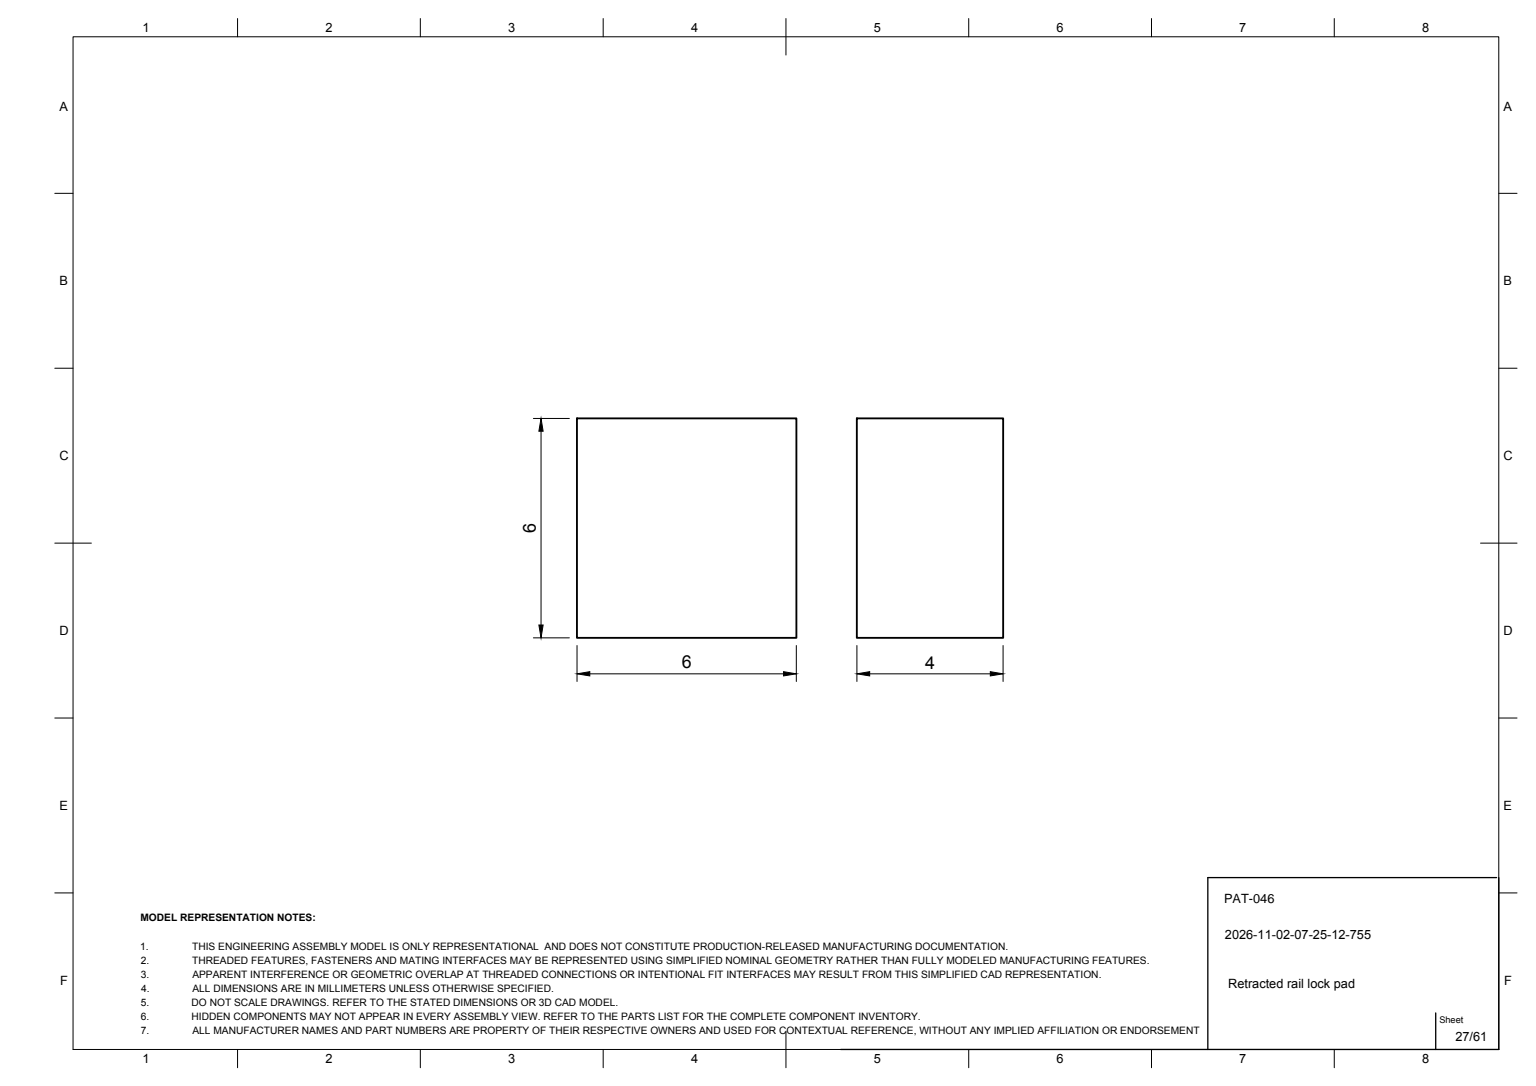
ISO-10303-21;
HEADER;
/* Generated by software containing ST-Developer
 * from STEP Tools, Inc. (www.steptools.com) 
 */

FILE_DESCRIPTION(
/* description */ ('Gear mesh backlash fixture'),
/* implementation_level */ '2;1');

FILE_NAME(
/* name */ 'Retracted rail lock pad.step',
/* time_stamp */ '2026-10-28T03:26:00-07:00',
/* author */ (''),
/* organization */ (''),
/* preprocessor_version */ 'ST-DEVELOPER v20.2',
/* originating_system */ 'Autodesk Translation Framework v15.17.0.0',
/* authorisation */ '');

FILE_SCHEMA (('AUTOMOTIVE_DESIGN { 1 0 10303 214 3 1 1 }'));
ENDSEC;

DATA;
#10=MECHANICAL_DESIGN_GEOMETRIC_PRESENTATION_REPRESENTATION('',(#1042),#57900);
#935=SHAPE_REPRESENTATION_RELATIONSHIP('SRR','None',#58132,#985);
#985=ADVANCED_BREP_SHAPE_REPRESENTATION('',(#1106),#57865);
#1042=STYLED_ITEM('',(#58479),#1106);
#1106=MANIFOLD_SOLID_BREP('Body1',#13603);
#1452=PLANE('',#14695);
#1453=PLANE('',#14696);
#1454=PLANE('',#14697);
#1455=PLANE('',#14698);
#1456=PLANE('',#14699);
#1457=PLANE('',#14700);
#1927=FACE_OUTER_BOUND('',#2795,.T.);
#1928=FACE_OUTER_BOUND('',#2796,.T.);
#1929=FACE_OUTER_BOUND('',#2797,.T.);
#1930=FACE_OUTER_BOUND('',#2798,.T.);
#1931=FACE_OUTER_BOUND('',#2799,.T.);
#1932=FACE_OUTER_BOUND('',#2800,.T.);
#2795=EDGE_LOOP('',(#9923,#9924,#9925,#9926));
#2796=EDGE_LOOP('',(#9927,#9928,#9929,#9930));
#2797=EDGE_LOOP('',(#9931,#9932,#9933,#9934));
#2798=EDGE_LOOP('',(#9935,#9936,#9937,#9938));
#2799=EDGE_LOOP('',(#9939,#9940,#9941,#9942));
#2800=EDGE_LOOP('',(#9943,#9944,#9945,#9946));
#3674=LINE('',#20759,#4563);
#3675=LINE('',#20761,#4564);
#3676=LINE('',#20763,#4565);
#3677=LINE('',#20764,#4566);
#3678=LINE('',#20767,#4567);
#3679=LINE('',#20769,#4568);
#3680=LINE('',#20770,#4569);
#3681=LINE('',#20773,#4570);
#3682=LINE('',#20775,#4571);
#3683=LINE('',#20776,#4572);
#3684=LINE('',#20778,#4573);
#3685=LINE('',#20779,#4574);
#4563=VECTOR('',#16843,1.);
#4564=VECTOR('',#16844,1.);
#4565=VECTOR('',#16845,1.);
#4566=VECTOR('',#16846,1.);
#4567=VECTOR('',#16849,1.);
#4568=VECTOR('',#16850,1.);
#4569=VECTOR('',#16851,1.);
#4570=VECTOR('',#16854,1.);
#4571=VECTOR('',#16855,1.);
#4572=VECTOR('',#16856,1.);
#4573=VECTOR('',#16859,1.);
#4574=VECTOR('',#16860,1.);
#6131=VERTEX_POINT('',#20757);
#6132=VERTEX_POINT('',#20758);
#6133=VERTEX_POINT('',#20760);
#6134=VERTEX_POINT('',#20762);
#6135=VERTEX_POINT('',#20766);
#6136=VERTEX_POINT('',#20768);
#6137=VERTEX_POINT('',#20772);
#6138=VERTEX_POINT('',#20774);
#7548=EDGE_CURVE('',#6131,#6132,#3674,.T.);
#7549=EDGE_CURVE('',#6132,#6133,#3675,.T.);
#7550=EDGE_CURVE('',#6134,#6133,#3676,.T.);
#7551=EDGE_CURVE('',#6131,#6134,#3677,.T.);
#7552=EDGE_CURVE('',#6135,#6131,#3678,.T.);
#7553=EDGE_CURVE('',#6136,#6134,#3679,.T.);
#7554=EDGE_CURVE('',#6135,#6136,#3680,.T.);
#7555=EDGE_CURVE('',#6137,#6135,#3681,.T.);
#7556=EDGE_CURVE('',#6138,#6136,#3682,.T.);
#7557=EDGE_CURVE('',#6137,#6138,#3683,.T.);
#7558=EDGE_CURVE('',#6132,#6137,#3684,.T.);
#7559=EDGE_CURVE('',#6133,#6138,#3685,.T.);
#9923=ORIENTED_EDGE('',*,*,#7548,.T.);
#9924=ORIENTED_EDGE('',*,*,#7549,.T.);
#9925=ORIENTED_EDGE('',*,*,#7550,.F.);
#9926=ORIENTED_EDGE('',*,*,#7551,.F.);
#9927=ORIENTED_EDGE('',*,*,#7552,.T.);
#9928=ORIENTED_EDGE('',*,*,#7551,.T.);
#9929=ORIENTED_EDGE('',*,*,#7553,.F.);
#9930=ORIENTED_EDGE('',*,*,#7554,.F.);
#9931=ORIENTED_EDGE('',*,*,#7555,.T.);
#9932=ORIENTED_EDGE('',*,*,#7554,.T.);
#9933=ORIENTED_EDGE('',*,*,#7556,.F.);
#9934=ORIENTED_EDGE('',*,*,#7557,.F.);
#9935=ORIENTED_EDGE('',*,*,#7558,.T.);
#9936=ORIENTED_EDGE('',*,*,#7557,.T.);
#9937=ORIENTED_EDGE('',*,*,#7559,.F.);
#9938=ORIENTED_EDGE('',*,*,#7549,.F.);
#9939=ORIENTED_EDGE('',*,*,#7559,.T.);
#9940=ORIENTED_EDGE('',*,*,#7556,.T.);
#9941=ORIENTED_EDGE('',*,*,#7553,.T.);
#9942=ORIENTED_EDGE('',*,*,#7550,.T.);
#9943=ORIENTED_EDGE('',*,*,#7558,.F.);
#9944=ORIENTED_EDGE('',*,*,#7548,.F.);
#9945=ORIENTED_EDGE('',*,*,#7552,.F.);
#9946=ORIENTED_EDGE('',*,*,#7555,.F.);
#13044=ADVANCED_FACE('',(#1927),#1452,.T.);
#13045=ADVANCED_FACE('',(#1928),#1453,.T.);
#13046=ADVANCED_FACE('',(#1929),#1454,.T.);
#13047=ADVANCED_FACE('',(#1930),#1455,.T.);
#13048=ADVANCED_FACE('',(#1931),#1456,.T.);
#13049=ADVANCED_FACE('',(#1932),#1457,.F.);
#13603=CLOSED_SHELL('',(#13044,#13045,#13046,#13047,#13048,#13049));
#14694=AXIS2_PLACEMENT_3D('',#20755,#16839,#16840);
#14695=AXIS2_PLACEMENT_3D('',#20756,#16841,#16842);
#14696=AXIS2_PLACEMENT_3D('',#20765,#16847,#16848);
#14697=AXIS2_PLACEMENT_3D('',#20771,#16852,#16853);
#14698=AXIS2_PLACEMENT_3D('',#20777,#16857,#16858);
#14699=AXIS2_PLACEMENT_3D('',#20780,#16861,#16862);
#14700=AXIS2_PLACEMENT_3D('',#20781,#16863,#16864);
#16839=DIRECTION('axis',(0.,0.,1.));
#16840=DIRECTION('refdir',(1.,0.,0.));
#16841=DIRECTION('center_axis',(0.,1.,0.));
#16842=DIRECTION('ref_axis',(-1.,0.,0.));
#16843=DIRECTION('',(-1.,0.,0.));
#16844=DIRECTION('',(0.,0.,1.));
#16845=DIRECTION('',(-1.,0.,0.));
#16846=DIRECTION('',(0.,0.,1.));
#16847=DIRECTION('center_axis',(1.,0.,0.));
#16848=DIRECTION('ref_axis',(0.,1.,0.));
#16849=DIRECTION('',(0.,1.,0.));
#16850=DIRECTION('',(0.,1.,0.));
#16851=DIRECTION('',(0.,0.,1.));
#16852=DIRECTION('center_axis',(0.,-1.,0.));
#16853=DIRECTION('ref_axis',(1.,0.,0.));
#16854=DIRECTION('',(1.,0.,0.));
#16855=DIRECTION('',(1.,0.,0.));
#16856=DIRECTION('',(0.,0.,1.));
#16857=DIRECTION('center_axis',(-1.,0.,0.));
#16858=DIRECTION('ref_axis',(0.,-1.,0.));
#16859=DIRECTION('',(0.,-1.,0.));
#16860=DIRECTION('',(0.,-1.,0.));
#16861=DIRECTION('center_axis',(0.,0.,1.));
#16862=DIRECTION('ref_axis',(1.,0.,0.));
#16863=DIRECTION('center_axis',(0.,0.,1.));
#16864=DIRECTION('ref_axis',(1.,0.,0.));
#20755=CARTESIAN_POINT('',(0.,0.,0.));
#20756=CARTESIAN_POINT('Origin',(9.8,7.2,0.8));
#20757=CARTESIAN_POINT('',(9.8,7.2,0.8));
#20758=CARTESIAN_POINT('',(9.2,7.2,0.8));
#20759=CARTESIAN_POINT('',(9.8,7.2,0.8));
#20760=CARTESIAN_POINT('',(9.2,7.2,1.4));
#20761=CARTESIAN_POINT('',(9.2,7.2,0.8));
#20762=CARTESIAN_POINT('',(9.8,7.2,1.4));
#20763=CARTESIAN_POINT('',(9.8,7.2,1.4));
#20764=CARTESIAN_POINT('',(9.8,7.2,0.8));
#20765=CARTESIAN_POINT('Origin',(9.8,6.8,0.8));
#20766=CARTESIAN_POINT('',(9.8,6.8,0.8));
#20767=CARTESIAN_POINT('',(9.8,6.8,0.8));
#20768=CARTESIAN_POINT('',(9.8,6.8,1.4));
#20769=CARTESIAN_POINT('',(9.8,6.8,1.4));
#20770=CARTESIAN_POINT('',(9.8,6.8,0.8));
#20771=CARTESIAN_POINT('Origin',(9.2,6.8,0.8));
#20772=CARTESIAN_POINT('',(9.2,6.8,0.8));
#20773=CARTESIAN_POINT('',(9.2,6.8,0.8));
#20774=CARTESIAN_POINT('',(9.2,6.8,1.4));
#20775=CARTESIAN_POINT('',(9.2,6.8,1.4));
#20776=CARTESIAN_POINT('',(9.2,6.8,0.8));
#20777=CARTESIAN_POINT('Origin',(9.2,7.2,0.8));
#20778=CARTESIAN_POINT('',(9.2,7.2,0.8));
#20779=CARTESIAN_POINT('',(9.2,7.2,1.4));
#20780=CARTESIAN_POINT('Origin',(9.5,7.,1.4));
#20781=CARTESIAN_POINT('Origin',(9.5,7.,0.8));
#57806=UNCERTAINTY_MEASURE_WITH_UNIT(LENGTH_MEASURE(0.001),#57901,
'DISTANCE_ACCURACY_VALUE',
'Maximum model space distance between geometric entities at asserted c
onnectivities');
#57841=UNCERTAINTY_MEASURE_WITH_UNIT(LENGTH_MEASURE(0.001),#57901,
'DISTANCE_ACCURACY_VALUE',
'Maximum model space distance between geometric entities at asserted c
onnectivities');
#57865=(
GEOMETRIC_REPRESENTATION_CONTEXT(3)
GLOBAL_UNCERTAINTY_ASSIGNED_CONTEXT((#57806))
GLOBAL_UNIT_ASSIGNED_CONTEXT((#57901,#57903,#57904))
REPRESENTATION_CONTEXT('','3D')
);
#57900=(
GEOMETRIC_REPRESENTATION_CONTEXT(3)
GLOBAL_UNCERTAINTY_ASSIGNED_CONTEXT((#57841))
GLOBAL_UNIT_ASSIGNED_CONTEXT((#57901,#57903,#57904))
REPRESENTATION_CONTEXT('','3D')
);
#57901=(
LENGTH_UNIT()
NAMED_UNIT(*)
SI_UNIT(.CENTI.,.METRE.)
);
#57903=(
NAMED_UNIT(*)
PLANE_ANGLE_UNIT()
SI_UNIT($,.RADIAN.)
);
#57904=(
NAMED_UNIT(*)
SI_UNIT($,.STERADIAN.)
SOLID_ANGLE_UNIT()
);
#57928=SHAPE_DEFINITION_REPRESENTATION(#57991,#58132);
#57991=PRODUCT_DEFINITION_SHAPE('',$,#58191);
#58132=SHAPE_REPRESENTATION('',(#14694),#57865);
#58167=PRODUCT_DEFINITION_CONTEXT('part definition',#58343,'design');
#58191=PRODUCT_DEFINITION('Retracted rail lock pad',
'Retracted rail lock pad',#58249,#58167);
#58249=PRODUCT_DEFINITION_FORMATION('',$,#58368);
#58343=APPLICATION_CONTEXT(
'Core Data for Automotive Mechanical Design Process');
#58344=PRODUCT_CONTEXT('part definition',#58343,'mechanical');
#58368=PRODUCT('Retracted rail lock pad','Retracted rail lock pad',
'Retracted rail lock pad',(#58344));
#58473=COLOUR_RGB('Off White',0.89,0.88,0.83);
#58474=FILL_AREA_STYLE_COLOUR('',#58473);
#58475=FILL_AREA_STYLE('',(#58474));
#58476=SURFACE_STYLE_FILL_AREA(#58475);
#58477=SURFACE_SIDE_STYLE('',(#58476));
#58478=SURFACE_STYLE_USAGE(.BOTH.,#58477);
#58479=PRESENTATION_STYLE_ASSIGNMENT((#58478));
ENDSEC;
END-ISO-10303-21;
